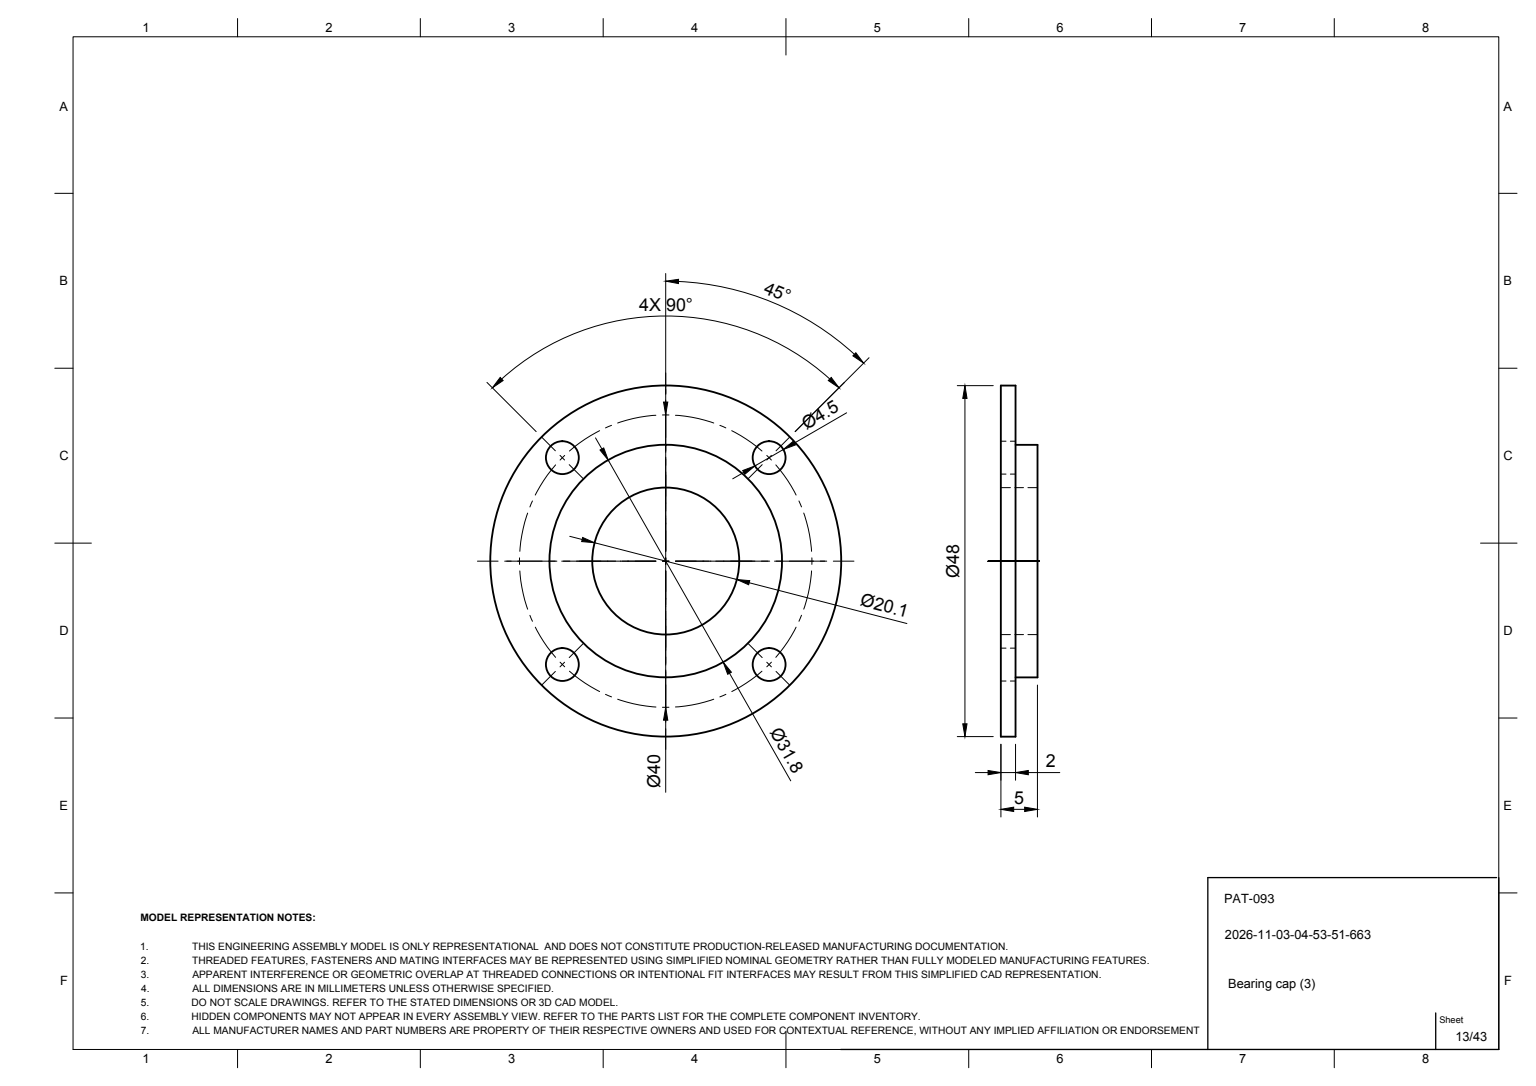
ISO-10303-21;
HEADER;
/* Generated by software containing ST-Developer
 * from STEP Tools, Inc. (www.steptools.com) 
 */

FILE_DESCRIPTION(
/* description */ ('Self-centering screw clamp'),
/* implementation_level */ '2;1');

FILE_NAME(
/* name */ 'Bearing cap (3).step',
/* time_stamp */ '2026-10-28T03:25:31-07:00',
/* author */ (''),
/* organization */ (''),
/* preprocessor_version */ 'ST-DEVELOPER v20.2',
/* originating_system */ 'Autodesk Translation Framework v15.17.0.0',
/* authorisation */ '');

FILE_SCHEMA (('AUTOMOTIVE_DESIGN { 1 0 10303 214 3 1 1 }'));
ENDSEC;

DATA;
#10=MECHANICAL_DESIGN_GEOMETRIC_PRESENTATION_REPRESENTATION('',(#636),#16799);
#554=SHAPE_REPRESENTATION_RELATIONSHIP('SRR','None',#17027,#595);
#595=ADVANCED_BREP_SHAPE_REPRESENTATION('',(#684),#16765);
#636=STYLED_ITEM('',(#17326),#684);
#684=MANIFOLD_SOLID_BREP('Body1',#9087);
#831=FACE_BOUND('',#2062,.T.);
#832=FACE_BOUND('',#2066,.T.);
#833=FACE_BOUND('',#2067,.T.);
#834=FACE_BOUND('',#2068,.T.);
#835=FACE_BOUND('',#2069,.T.);
#836=FACE_BOUND('',#2070,.T.);
#837=FACE_BOUND('',#2072,.T.);
#838=FACE_BOUND('',#2073,.T.);
#839=FACE_BOUND('',#2074,.T.);
#840=FACE_BOUND('',#2075,.T.);
#841=FACE_BOUND('',#2076,.T.);
#1101=PLANE('',#9935);
#1102=PLANE('',#9942);
#1103=PLANE('',#9943);
#1439=FACE_OUTER_BOUND('',#2056,.T.);
#1440=FACE_OUTER_BOUND('',#2057,.T.);
#1441=FACE_OUTER_BOUND('',#2058,.T.);
#1442=FACE_OUTER_BOUND('',#2059,.T.);
#1443=FACE_OUTER_BOUND('',#2060,.T.);
#1444=FACE_OUTER_BOUND('',#2061,.T.);
#1445=FACE_OUTER_BOUND('',#2063,.T.);
#1446=FACE_OUTER_BOUND('',#2064,.T.);
#1447=FACE_OUTER_BOUND('',#2065,.T.);
#1448=FACE_OUTER_BOUND('',#2071,.T.);
#2056=EDGE_LOOP('',(#6937,#6938,#6939,#6940));
#2057=EDGE_LOOP('',(#6941,#6942,#6943,#6944));
#2058=EDGE_LOOP('',(#6945,#6946,#6947,#6948));
#2059=EDGE_LOOP('',(#6949,#6950,#6951,#6952));
#2060=EDGE_LOOP('',(#6953,#6954,#6955,#6956));
#2061=EDGE_LOOP('',(#6957));
#2062=EDGE_LOOP('',(#6958));
#2063=EDGE_LOOP('',(#6959,#6960,#6961,#6962));
#2064=EDGE_LOOP('',(#6963,#6964,#6965,#6966));
#2065=EDGE_LOOP('',(#6967));
#2066=EDGE_LOOP('',(#6968));
#2067=EDGE_LOOP('',(#6969));
#2068=EDGE_LOOP('',(#6970));
#2069=EDGE_LOOP('',(#6971));
#2070=EDGE_LOOP('',(#6972));
#2071=EDGE_LOOP('',(#6973));
#2072=EDGE_LOOP('',(#6974));
#2073=EDGE_LOOP('',(#6975));
#2074=EDGE_LOOP('',(#6976));
#2075=EDGE_LOOP('',(#6977));
#2076=EDGE_LOOP('',(#6978));
#2816=LINE('',#14623,#3389);
#2817=LINE('',#14629,#3390);
#2818=LINE('',#14635,#3391);
#2819=LINE('',#14641,#3392);
#2820=LINE('',#14647,#3393);
#2821=LINE('',#14655,#3394);
#2822=LINE('',#14660,#3395);
#3389=VECTOR('',#11681,0.225);
#3390=VECTOR('',#11688,0.225);
#3391=VECTOR('',#11695,0.225);
#3392=VECTOR('',#11702,0.225);
#3393=VECTOR('',#11709,1.59);
#3394=VECTOR('',#11720,1.005);
#3395=VECTOR('',#11725,2.4);
#3885=CIRCLE('',#9921,0.225);
#3886=CIRCLE('',#9922,0.225);
#3887=CIRCLE('',#9924,0.225);
#3888=CIRCLE('',#9925,0.225);
#3889=CIRCLE('',#9927,0.225);
#3890=CIRCLE('',#9928,0.225);
#3891=CIRCLE('',#9930,0.225);
#3892=CIRCLE('',#9931,0.225);
#3893=CIRCLE('',#9933,1.59);
#3894=CIRCLE('',#9934,1.59);
#3895=CIRCLE('',#9936,1.005);
#3896=CIRCLE('',#9938,1.005);
#3897=CIRCLE('',#9940,2.4);
#3898=CIRCLE('',#9941,2.4);
#4499=VERTEX_POINT('',#14620);
#4500=VERTEX_POINT('',#14622);
#4501=VERTEX_POINT('',#14626);
#4502=VERTEX_POINT('',#14628);
#4503=VERTEX_POINT('',#14632);
#4504=VERTEX_POINT('',#14634);
#4505=VERTEX_POINT('',#14638);
#4506=VERTEX_POINT('',#14640);
#4507=VERTEX_POINT('',#14644);
#4508=VERTEX_POINT('',#14646);
#4509=VERTEX_POINT('',#14650);
#4510=VERTEX_POINT('',#14653);
#4511=VERTEX_POINT('',#14657);
#4512=VERTEX_POINT('',#14659);
#5393=EDGE_CURVE('',#4499,#4499,#3885,.T.);
#5394=EDGE_CURVE('',#4499,#4500,#2816,.T.);
#5395=EDGE_CURVE('',#4500,#4500,#3886,.T.);
#5396=EDGE_CURVE('',#4501,#4501,#3887,.T.);
#5397=EDGE_CURVE('',#4501,#4502,#2817,.T.);
#5398=EDGE_CURVE('',#4502,#4502,#3888,.T.);
#5399=EDGE_CURVE('',#4503,#4503,#3889,.T.);
#5400=EDGE_CURVE('',#4503,#4504,#2818,.T.);
#5401=EDGE_CURVE('',#4504,#4504,#3890,.T.);
#5402=EDGE_CURVE('',#4505,#4505,#3891,.T.);
#5403=EDGE_CURVE('',#4505,#4506,#2819,.T.);
#5404=EDGE_CURVE('',#4506,#4506,#3892,.T.);
#5405=EDGE_CURVE('',#4507,#4507,#3893,.T.);
#5406=EDGE_CURVE('',#4507,#4508,#2820,.T.);
#5407=EDGE_CURVE('',#4508,#4508,#3894,.T.);
#5408=EDGE_CURVE('',#4509,#4509,#3895,.T.);
#5409=EDGE_CURVE('',#4510,#4510,#3896,.T.);
#5410=EDGE_CURVE('',#4510,#4509,#2821,.T.);
#5411=EDGE_CURVE('',#4511,#4511,#3897,.T.);
#5412=EDGE_CURVE('',#4511,#4512,#2822,.T.);
#5413=EDGE_CURVE('',#4512,#4512,#3898,.T.);
#6937=ORIENTED_EDGE('',*,*,#5393,.F.);
#6938=ORIENTED_EDGE('',*,*,#5394,.T.);
#6939=ORIENTED_EDGE('',*,*,#5395,.F.);
#6940=ORIENTED_EDGE('',*,*,#5394,.F.);
#6941=ORIENTED_EDGE('',*,*,#5396,.F.);
#6942=ORIENTED_EDGE('',*,*,#5397,.T.);
#6943=ORIENTED_EDGE('',*,*,#5398,.F.);
#6944=ORIENTED_EDGE('',*,*,#5397,.F.);
#6945=ORIENTED_EDGE('',*,*,#5399,.F.);
#6946=ORIENTED_EDGE('',*,*,#5400,.T.);
#6947=ORIENTED_EDGE('',*,*,#5401,.F.);
#6948=ORIENTED_EDGE('',*,*,#5400,.F.);
#6949=ORIENTED_EDGE('',*,*,#5402,.F.);
#6950=ORIENTED_EDGE('',*,*,#5403,.T.);
#6951=ORIENTED_EDGE('',*,*,#5404,.F.);
#6952=ORIENTED_EDGE('',*,*,#5403,.F.);
#6953=ORIENTED_EDGE('',*,*,#5405,.F.);
#6954=ORIENTED_EDGE('',*,*,#5406,.T.);
#6955=ORIENTED_EDGE('',*,*,#5407,.T.);
#6956=ORIENTED_EDGE('',*,*,#5406,.F.);
#6957=ORIENTED_EDGE('',*,*,#5407,.F.);
#6958=ORIENTED_EDGE('',*,*,#5408,.F.);
#6959=ORIENTED_EDGE('',*,*,#5409,.F.);
#6960=ORIENTED_EDGE('',*,*,#5410,.T.);
#6961=ORIENTED_EDGE('',*,*,#5408,.T.);
#6962=ORIENTED_EDGE('',*,*,#5410,.F.);
#6963=ORIENTED_EDGE('',*,*,#5411,.F.);
#6964=ORIENTED_EDGE('',*,*,#5412,.T.);
#6965=ORIENTED_EDGE('',*,*,#5413,.T.);
#6966=ORIENTED_EDGE('',*,*,#5412,.F.);
#6967=ORIENTED_EDGE('',*,*,#5411,.T.);
#6968=ORIENTED_EDGE('',*,*,#5409,.T.);
#6969=ORIENTED_EDGE('',*,*,#5404,.T.);
#6970=ORIENTED_EDGE('',*,*,#5401,.T.);
#6971=ORIENTED_EDGE('',*,*,#5398,.T.);
#6972=ORIENTED_EDGE('',*,*,#5395,.T.);
#6973=ORIENTED_EDGE('',*,*,#5413,.F.);
#6974=ORIENTED_EDGE('',*,*,#5405,.T.);
#6975=ORIENTED_EDGE('',*,*,#5402,.T.);
#6976=ORIENTED_EDGE('',*,*,#5399,.T.);
#6977=ORIENTED_EDGE('',*,*,#5396,.T.);
#6978=ORIENTED_EDGE('',*,*,#5393,.T.);
#8436=CYLINDRICAL_SURFACE('',#9920,0.225);
#8437=CYLINDRICAL_SURFACE('',#9923,0.225);
#8438=CYLINDRICAL_SURFACE('',#9926,0.225);
#8439=CYLINDRICAL_SURFACE('',#9929,0.225);
#8440=CYLINDRICAL_SURFACE('',#9932,1.59);
#8441=CYLINDRICAL_SURFACE('',#9937,1.005);
#8442=CYLINDRICAL_SURFACE('',#9939,2.4);
#8737=ADVANCED_FACE('',(#1439),#8436,.F.);
#8738=ADVANCED_FACE('',(#1440),#8437,.F.);
#8739=ADVANCED_FACE('',(#1441),#8438,.F.);
#8740=ADVANCED_FACE('',(#1442),#8439,.F.);
#8741=ADVANCED_FACE('',(#1443),#8440,.T.);
#8742=ADVANCED_FACE('',(#1444,#831),#1101,.F.);
#8743=ADVANCED_FACE('',(#1445),#8441,.F.);
#8744=ADVANCED_FACE('',(#1446),#8442,.T.);
#8745=ADVANCED_FACE('',(#1447,#832,#833,#834,#835,#836),#1102,.T.);
#8746=ADVANCED_FACE('',(#1448,#837,#838,#839,#840,#841),#1103,.F.);
#9087=CLOSED_SHELL('',(#8737,#8738,#8739,#8740,#8741,#8742,#8743,#8744,
#8745,#8746));
#9919=AXIS2_PLACEMENT_3D('',#14618,#11675,#11676);
#9920=AXIS2_PLACEMENT_3D('',#14619,#11677,#11678);
#9921=AXIS2_PLACEMENT_3D('',#14621,#11679,#11680);
#9922=AXIS2_PLACEMENT_3D('',#14624,#11682,#11683);
#9923=AXIS2_PLACEMENT_3D('',#14625,#11684,#11685);
#9924=AXIS2_PLACEMENT_3D('',#14627,#11686,#11687);
#9925=AXIS2_PLACEMENT_3D('',#14630,#11689,#11690);
#9926=AXIS2_PLACEMENT_3D('',#14631,#11691,#11692);
#9927=AXIS2_PLACEMENT_3D('',#14633,#11693,#11694);
#9928=AXIS2_PLACEMENT_3D('',#14636,#11696,#11697);
#9929=AXIS2_PLACEMENT_3D('',#14637,#11698,#11699);
#9930=AXIS2_PLACEMENT_3D('',#14639,#11700,#11701);
#9931=AXIS2_PLACEMENT_3D('',#14642,#11703,#11704);
#9932=AXIS2_PLACEMENT_3D('',#14643,#11705,#11706);
#9933=AXIS2_PLACEMENT_3D('',#14645,#11707,#11708);
#9934=AXIS2_PLACEMENT_3D('',#14648,#11710,#11711);
#9935=AXIS2_PLACEMENT_3D('',#14649,#11712,#11713);
#9936=AXIS2_PLACEMENT_3D('',#14651,#11714,#11715);
#9937=AXIS2_PLACEMENT_3D('',#14652,#11716,#11717);
#9938=AXIS2_PLACEMENT_3D('',#14654,#11718,#11719);
#9939=AXIS2_PLACEMENT_3D('',#14656,#11721,#11722);
#9940=AXIS2_PLACEMENT_3D('',#14658,#11723,#11724);
#9941=AXIS2_PLACEMENT_3D('',#14661,#11726,#11727);
#9942=AXIS2_PLACEMENT_3D('',#14662,#11728,#11729);
#9943=AXIS2_PLACEMENT_3D('',#14663,#11730,#11731);
#11675=DIRECTION('axis',(0.,0.,1.));
#11676=DIRECTION('refdir',(1.,0.,0.));
#11677=DIRECTION('center_axis',(1.,0.,0.));
#11678=DIRECTION('ref_axis',(0.,0.,-1.));
#11679=DIRECTION('center_axis',(1.,0.,0.));
#11680=DIRECTION('ref_axis',(0.,0.,-1.));
#11681=DIRECTION('',(1.,0.,0.));
#11682=DIRECTION('center_axis',(-1.,0.,0.));
#11683=DIRECTION('ref_axis',(0.,0.,-1.));
#11684=DIRECTION('center_axis',(1.,0.,0.));
#11685=DIRECTION('ref_axis',(0.,0.,-1.));
#11686=DIRECTION('center_axis',(1.,0.,0.));
#11687=DIRECTION('ref_axis',(0.,0.,-1.));
#11688=DIRECTION('',(1.,0.,0.));
#11689=DIRECTION('center_axis',(-1.,0.,0.));
#11690=DIRECTION('ref_axis',(0.,0.,-1.));
#11691=DIRECTION('center_axis',(1.,0.,0.));
#11692=DIRECTION('ref_axis',(0.,0.,-1.));
#11693=DIRECTION('center_axis',(1.,0.,0.));
#11694=DIRECTION('ref_axis',(0.,0.,-1.));
#11695=DIRECTION('',(1.,0.,0.));
#11696=DIRECTION('center_axis',(-1.,0.,0.));
#11697=DIRECTION('ref_axis',(0.,0.,-1.));
#11698=DIRECTION('center_axis',(1.,0.,0.));
#11699=DIRECTION('ref_axis',(0.,0.,-1.));
#11700=DIRECTION('center_axis',(1.,0.,0.));
#11701=DIRECTION('ref_axis',(0.,0.,-1.));
#11702=DIRECTION('',(1.,0.,0.));
#11703=DIRECTION('center_axis',(-1.,0.,0.));
#11704=DIRECTION('ref_axis',(0.,0.,-1.));
#11705=DIRECTION('center_axis',(1.,0.,0.));
#11706=DIRECTION('ref_axis',(0.,0.,-1.));
#11707=DIRECTION('center_axis',(1.,0.,0.));
#11708=DIRECTION('ref_axis',(0.,0.,-1.));
#11709=DIRECTION('',(-1.,0.,0.));
#11710=DIRECTION('center_axis',(1.,0.,0.));
#11711=DIRECTION('ref_axis',(0.,0.,-1.));
#11712=DIRECTION('center_axis',(1.,0.,0.));
#11713=DIRECTION('ref_axis',(0.,0.,-1.));
#11714=DIRECTION('center_axis',(-1.,0.,0.));
#11715=DIRECTION('ref_axis',(0.,0.,-1.));
#11716=DIRECTION('center_axis',(1.,0.,0.));
#11717=DIRECTION('ref_axis',(0.,0.,-1.));
#11718=DIRECTION('center_axis',(-1.,0.,0.));
#11719=DIRECTION('ref_axis',(0.,0.,-1.));
#11720=DIRECTION('',(-1.,0.,0.));
#11721=DIRECTION('center_axis',(1.,0.,0.));
#11722=DIRECTION('ref_axis',(0.,0.,-1.));
#11723=DIRECTION('center_axis',(1.,0.,0.));
#11724=DIRECTION('ref_axis',(0.,0.,-1.));
#11725=DIRECTION('',(-1.,0.,0.));
#11726=DIRECTION('center_axis',(1.,0.,0.));
#11727=DIRECTION('ref_axis',(0.,0.,-1.));
#11728=DIRECTION('center_axis',(1.,0.,0.));
#11729=DIRECTION('ref_axis',(0.,0.,-1.));
#11730=DIRECTION('center_axis',(1.,0.,0.));
#11731=DIRECTION('ref_axis',(0.,0.,-1.));
#14618=CARTESIAN_POINT('',(0.,0.,0.));
#14619=CARTESIAN_POINT('Origin',(12.2,-1.4142135623731,2.58578643762691));
#14620=CARTESIAN_POINT('',(12.3,-1.4142135623731,2.81078643762691));
#14621=CARTESIAN_POINT('Origin',(12.3,-1.4142135623731,2.58578643762691));
#14622=CARTESIAN_POINT('',(12.5,-1.4142135623731,2.81078643762691));
#14623=CARTESIAN_POINT('',(12.2,-1.4142135623731,2.81078643762691));
#14624=CARTESIAN_POINT('Origin',(12.5,-1.4142135623731,2.58578643762691));
#14625=CARTESIAN_POINT('Origin',(12.2,-1.41421356237309,5.41421356237309));
#14626=CARTESIAN_POINT('',(12.3,-1.41421356237309,5.63921356237309));
#14627=CARTESIAN_POINT('Origin',(12.3,-1.41421356237309,5.41421356237309));
#14628=CARTESIAN_POINT('',(12.5,-1.41421356237309,5.63921356237309));
#14629=CARTESIAN_POINT('',(12.2,-1.41421356237309,5.63921356237309));
#14630=CARTESIAN_POINT('Origin',(12.5,-1.41421356237309,5.41421356237309));
#14631=CARTESIAN_POINT('Origin',(12.2,1.4142135623731,5.41421356237309));
#14632=CARTESIAN_POINT('',(12.3,1.4142135623731,5.63921356237309));
#14633=CARTESIAN_POINT('Origin',(12.3,1.4142135623731,5.41421356237309));
#14634=CARTESIAN_POINT('',(12.5,1.4142135623731,5.63921356237309));
#14635=CARTESIAN_POINT('',(12.2,1.4142135623731,5.63921356237309));
#14636=CARTESIAN_POINT('Origin',(12.5,1.4142135623731,5.41421356237309));
#14637=CARTESIAN_POINT('Origin',(12.2,1.41421356237309,2.5857864376269));
#14638=CARTESIAN_POINT('',(12.3,1.41421356237309,2.8107864376269));
#14639=CARTESIAN_POINT('Origin',(12.3,1.41421356237309,2.5857864376269));
#14640=CARTESIAN_POINT('',(12.5,1.41421356237309,2.8107864376269));
#14641=CARTESIAN_POINT('',(12.2,1.41421356237309,2.8107864376269));
#14642=CARTESIAN_POINT('Origin',(12.5,1.41421356237309,2.5857864376269));
#14643=CARTESIAN_POINT('Origin',(12.,0.,4.));
#14644=CARTESIAN_POINT('',(12.3,-1.94718841064429E-16,5.59));
#14645=CARTESIAN_POINT('Origin',(12.3,0.,4.));
#14646=CARTESIAN_POINT('',(12.,-1.94718841064429E-16,5.59));
#14647=CARTESIAN_POINT('',(12.,-1.94718841064429E-16,5.59));
#14648=CARTESIAN_POINT('Origin',(12.,0.,4.));
#14649=CARTESIAN_POINT('Origin',(12.,0.,4.));
#14650=CARTESIAN_POINT('',(12.,-1.23077003314309E-16,5.005));
#14651=CARTESIAN_POINT('Origin',(12.,0.,4.));
#14652=CARTESIAN_POINT('Origin',(12.3,0.,4.));
#14653=CARTESIAN_POINT('',(12.5,-1.23077003314309E-16,5.005));
#14654=CARTESIAN_POINT('Origin',(12.5,0.,4.));
#14655=CARTESIAN_POINT('',(12.3,-1.23077003314309E-16,5.005));
#14656=CARTESIAN_POINT('Origin',(12.3,0.,4.));
#14657=CARTESIAN_POINT('',(12.5,-2.93915231795365E-16,6.4));
#14658=CARTESIAN_POINT('Origin',(12.5,0.,4.));
#14659=CARTESIAN_POINT('',(12.3,-2.93915231795365E-16,6.4));
#14660=CARTESIAN_POINT('',(12.3,-2.93915231795365E-16,6.4));
#14661=CARTESIAN_POINT('Origin',(12.3,0.,4.));
#14662=CARTESIAN_POINT('Origin',(12.5,0.,4.));
#14663=CARTESIAN_POINT('Origin',(12.3,0.,4.));
#16716=UNCERTAINTY_MEASURE_WITH_UNIT(LENGTH_MEASURE(0.001),#16800,
'DISTANCE_ACCURACY_VALUE',
'Maximum model space distance between geometric entities at asserted c
onnectivities');
#16750=UNCERTAINTY_MEASURE_WITH_UNIT(LENGTH_MEASURE(0.001),#16800,
'DISTANCE_ACCURACY_VALUE',
'Maximum model space distance between geometric entities at asserted c
onnectivities');
#16765=(
GEOMETRIC_REPRESENTATION_CONTEXT(3)
GLOBAL_UNCERTAINTY_ASSIGNED_CONTEXT((#16716))
GLOBAL_UNIT_ASSIGNED_CONTEXT((#16800,#16802,#16803))
REPRESENTATION_CONTEXT('','3D')
);
#16799=(
GEOMETRIC_REPRESENTATION_CONTEXT(3)
GLOBAL_UNCERTAINTY_ASSIGNED_CONTEXT((#16750))
GLOBAL_UNIT_ASSIGNED_CONTEXT((#16800,#16802,#16803))
REPRESENTATION_CONTEXT('','3D')
);
#16800=(
LENGTH_UNIT()
NAMED_UNIT(*)
SI_UNIT(.CENTI.,.METRE.)
);
#16802=(
NAMED_UNIT(*)
PLANE_ANGLE_UNIT()
SI_UNIT($,.RADIAN.)
);
#16803=(
NAMED_UNIT(*)
SI_UNIT($,.STERADIAN.)
SOLID_ANGLE_UNIT()
);
#16818=SHAPE_DEFINITION_REPRESENTATION(#16866,#17027);
#16866=PRODUCT_DEFINITION_SHAPE('',$,#17076);
#17027=SHAPE_REPRESENTATION('',(#9919),#16765);
#17061=PRODUCT_DEFINITION_CONTEXT('part definition',#17207,'design');
#17076=PRODUCT_DEFINITION('Bearing cap (3)','Bearing cap (3)',#17124,#17061);
#17124=PRODUCT_DEFINITION_FORMATION('',$,#17223);
#17207=APPLICATION_CONTEXT(
'Core Data for Automotive Mechanical Design Process');
#17208=PRODUCT_CONTEXT('part definition',#17207,'mechanical');
#17223=PRODUCT('Bearing cap (3)','Bearing cap (3)','Bearing cap (3)',(#17208));
#17320=COLOUR_RGB('Grey',0.48,0.52,0.57);
#17321=FILL_AREA_STYLE_COLOUR('',#17320);
#17322=FILL_AREA_STYLE('',(#17321));
#17323=SURFACE_STYLE_FILL_AREA(#17322);
#17324=SURFACE_SIDE_STYLE('',(#17323));
#17325=SURFACE_STYLE_USAGE(.BOTH.,#17324);
#17326=PRESENTATION_STYLE_ASSIGNMENT((#17325));
ENDSEC;
END-ISO-10303-21;
